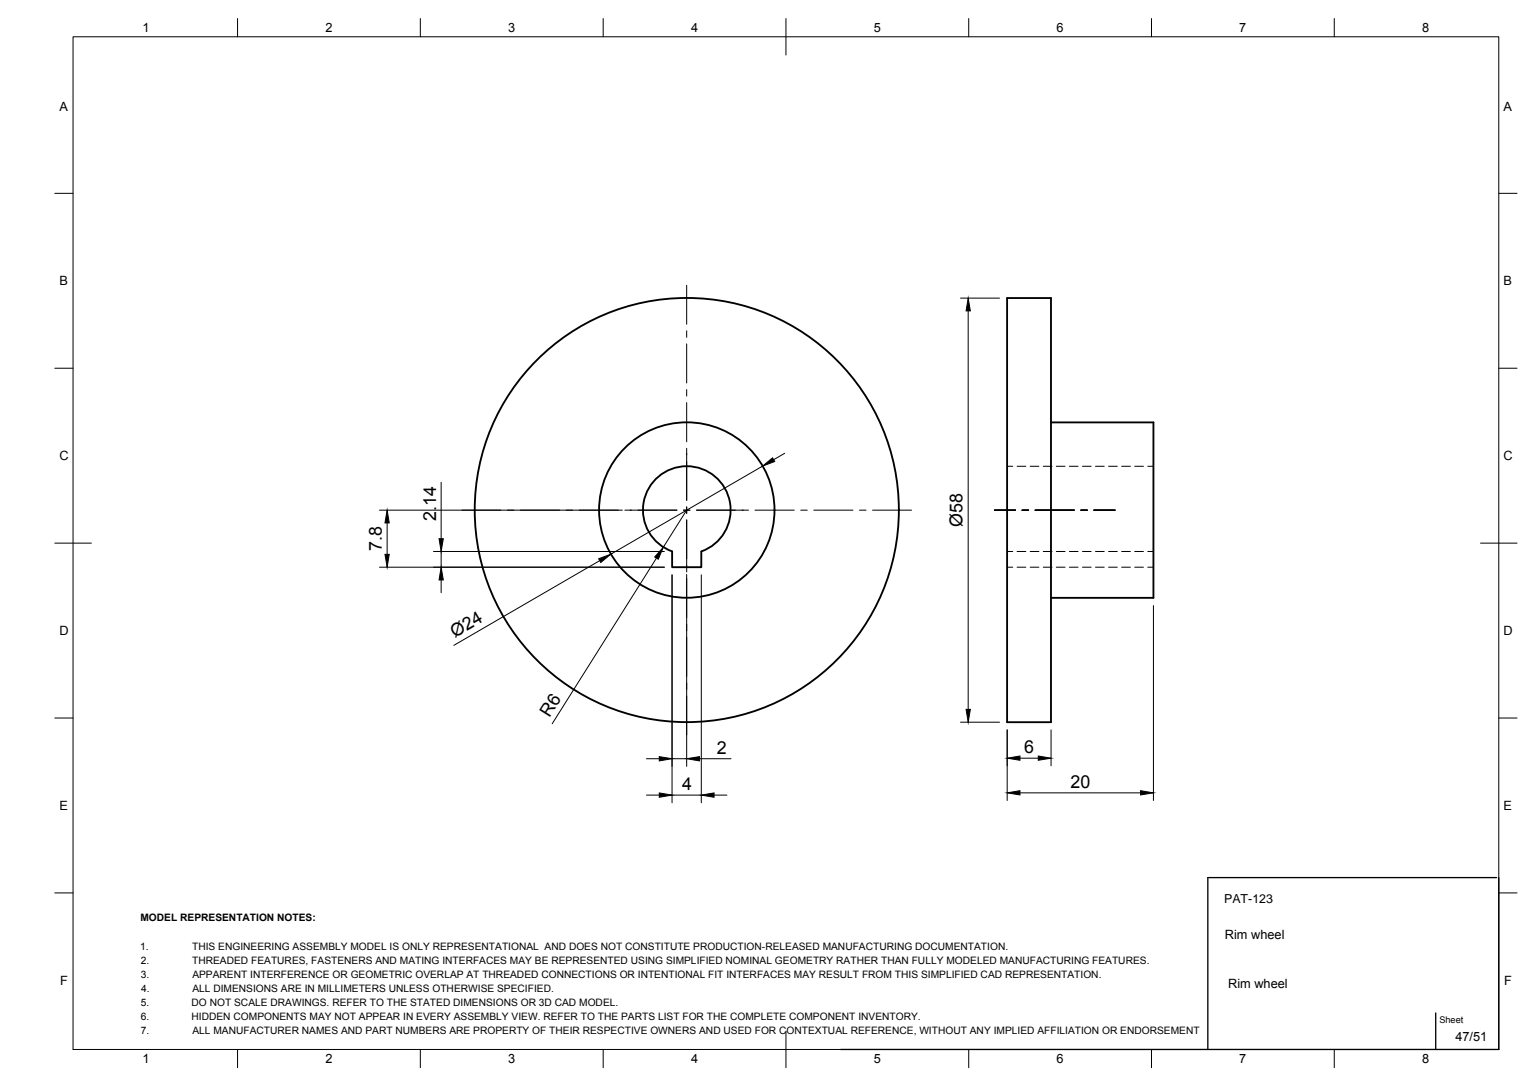
ISO-10303-21;
HEADER;
/* Generated by software containing ST-Developer
 * from STEP Tools, Inc. (www.steptools.com) 
 */

FILE_DESCRIPTION(
/* description */ ('Worm-less right-angle friction wheel drive'),
/* implementation_level */ '2;1');

FILE_NAME(
/* name */ 'Rim wheel.step',
/* time_stamp */ '2026-10-28T03:22:36-07:00',
/* author */ (''),
/* organization */ (''),
/* preprocessor_version */ 'ST-DEVELOPER v20.2',
/* originating_system */ 'Autodesk Translation Framework v15.17.0.0',
/* authorisation */ '');

FILE_SCHEMA (('AUTOMOTIVE_DESIGN { 1 0 10303 214 3 1 1 }'));
ENDSEC;

DATA;
#10=MECHANICAL_DESIGN_GEOMETRIC_PRESENTATION_REPRESENTATION('',(#658),#17046);
#557=SHAPE_REPRESENTATION_RELATIONSHIP('SRR','None',#17303,#604);
#604=ADVANCED_BREP_SHAPE_REPRESENTATION('',(#708),#17039);
#658=STYLED_ITEM('',(#17584),#708);
#708=MANIFOLD_SOLID_BREP('Body1',#8217);
#940=FACE_BOUND('',#2317,.T.);
#941=FACE_BOUND('',#2320,.T.);
#942=FACE_BOUND('',#2324,.T.);
#1171=PLANE('',#9665);
#1172=PLANE('',#9666);
#1173=PLANE('',#9667);
#1174=PLANE('',#9668);
#1175=PLANE('',#9673);
#1176=PLANE('',#9679);
#1622=FACE_OUTER_BOUND('',#2313,.T.);
#1623=FACE_OUTER_BOUND('',#2314,.T.);
#1624=FACE_OUTER_BOUND('',#2315,.T.);
#1625=FACE_OUTER_BOUND('',#2316,.T.);
#1626=FACE_OUTER_BOUND('',#2318,.T.);
#1627=FACE_OUTER_BOUND('',#2319,.T.);
#1628=FACE_OUTER_BOUND('',#2321,.T.);
#1629=FACE_OUTER_BOUND('',#2322,.T.);
#1630=FACE_OUTER_BOUND('',#2323,.T.);
#2313=EDGE_LOOP('',(#7296,#7297,#7298,#7299));
#2314=EDGE_LOOP('',(#7300,#7301,#7302,#7303));
#2315=EDGE_LOOP('',(#7304,#7305,#7306,#7307));
#2316=EDGE_LOOP('',(#7308));
#2317=EDGE_LOOP('',(#7309,#7310,#7311,#7312));
#2318=EDGE_LOOP('',(#7313,#7314,#7315,#7316));
#2319=EDGE_LOOP('',(#7317));
#2320=EDGE_LOOP('',(#7318));
#2321=EDGE_LOOP('',(#7319,#7320,#7321,#7322));
#2322=EDGE_LOOP('',(#7323,#7324,#7325,#7326));
#2323=EDGE_LOOP('',(#7327));
#2324=EDGE_LOOP('',(#7328,#7329,#7330,#7331));
#2843=LINE('',#16561,#3383);
#2844=LINE('',#16563,#3384);
#2845=LINE('',#16565,#3385);
#2846=LINE('',#16566,#3386);
#2847=LINE('',#16569,#3387);
#2848=LINE('',#16571,#3388);
#2849=LINE('',#16572,#3389);
#2850=LINE('',#16575,#3390);
#2851=LINE('',#16577,#3391);
#2852=LINE('',#16578,#3392);
#2853=LINE('',#16592,#3393);
#2854=LINE('',#16595,#3394);
#3383=VECTOR('',#12087,1.);
#3384=VECTOR('',#12088,1.);
#3385=VECTOR('',#12089,1.);
#3386=VECTOR('',#12090,1.);
#3387=VECTOR('',#12093,1.);
#3388=VECTOR('',#12094,1.);
#3389=VECTOR('',#12095,1.);
#3390=VECTOR('',#12098,1.);
#3391=VECTOR('',#12099,1.);
#3392=VECTOR('',#12100,1.);
#3393=VECTOR('',#12119,2.9);
#3394=VECTOR('',#12124,1.2);
#3840=CIRCLE('',#9669,1.2);
#3841=CIRCLE('',#9670,0.6);
#3842=CIRCLE('',#9672,0.6);
#3843=CIRCLE('',#9674,2.9);
#3844=CIRCLE('',#9675,1.2);
#3845=CIRCLE('',#9677,2.9);
#4459=VERTEX_POINT('',#16559);
#4460=VERTEX_POINT('',#16560);
#4461=VERTEX_POINT('',#16562);
#4462=VERTEX_POINT('',#16564);
#4463=VERTEX_POINT('',#16568);
#4464=VERTEX_POINT('',#16570);
#4465=VERTEX_POINT('',#16574);
#4466=VERTEX_POINT('',#16576);
#4467=VERTEX_POINT('',#16580);
#4468=VERTEX_POINT('',#16586);
#4469=VERTEX_POINT('',#16588);
#4470=VERTEX_POINT('',#16591);
#5417=EDGE_CURVE('',#4459,#4460,#2843,.T.);
#5418=EDGE_CURVE('',#4459,#4461,#2844,.T.);
#5419=EDGE_CURVE('',#4462,#4461,#2845,.T.);
#5420=EDGE_CURVE('',#4460,#4462,#2846,.T.);
#5421=EDGE_CURVE('',#4463,#4459,#2847,.T.);
#5422=EDGE_CURVE('',#4463,#4464,#2848,.T.);
#5423=EDGE_CURVE('',#4461,#4464,#2849,.T.);
#5424=EDGE_CURVE('',#4465,#4463,#2850,.T.);
#5425=EDGE_CURVE('',#4466,#4465,#2851,.T.);
#5426=EDGE_CURVE('',#4464,#4466,#2852,.T.);
#5427=EDGE_CURVE('',#4467,#4467,#3840,.T.);
#5428=EDGE_CURVE('',#4466,#4462,#3841,.T.);
#5429=EDGE_CURVE('',#4465,#4460,#3842,.T.);
#5430=EDGE_CURVE('',#4468,#4468,#3843,.T.);
#5431=EDGE_CURVE('',#4469,#4469,#3844,.T.);
#5432=EDGE_CURVE('',#4468,#4470,#2853,.T.);
#5433=EDGE_CURVE('',#4470,#4470,#3845,.T.);
#5434=EDGE_CURVE('',#4467,#4469,#2854,.T.);
#7296=ORIENTED_EDGE('',*,*,#5417,.F.);
#7297=ORIENTED_EDGE('',*,*,#5418,.T.);
#7298=ORIENTED_EDGE('',*,*,#5419,.F.);
#7299=ORIENTED_EDGE('',*,*,#5420,.F.);
#7300=ORIENTED_EDGE('',*,*,#5421,.F.);
#7301=ORIENTED_EDGE('',*,*,#5422,.T.);
#7302=ORIENTED_EDGE('',*,*,#5423,.F.);
#7303=ORIENTED_EDGE('',*,*,#5418,.F.);
#7304=ORIENTED_EDGE('',*,*,#5424,.F.);
#7305=ORIENTED_EDGE('',*,*,#5425,.F.);
#7306=ORIENTED_EDGE('',*,*,#5426,.F.);
#7307=ORIENTED_EDGE('',*,*,#5422,.F.);
#7308=ORIENTED_EDGE('',*,*,#5427,.T.);
#7309=ORIENTED_EDGE('',*,*,#5419,.T.);
#7310=ORIENTED_EDGE('',*,*,#5423,.T.);
#7311=ORIENTED_EDGE('',*,*,#5426,.T.);
#7312=ORIENTED_EDGE('',*,*,#5428,.T.);
#7313=ORIENTED_EDGE('',*,*,#5420,.T.);
#7314=ORIENTED_EDGE('',*,*,#5428,.F.);
#7315=ORIENTED_EDGE('',*,*,#5425,.T.);
#7316=ORIENTED_EDGE('',*,*,#5429,.T.);
#7317=ORIENTED_EDGE('',*,*,#5430,.T.);
#7318=ORIENTED_EDGE('',*,*,#5431,.F.);
#7319=ORIENTED_EDGE('',*,*,#5430,.F.);
#7320=ORIENTED_EDGE('',*,*,#5432,.T.);
#7321=ORIENTED_EDGE('',*,*,#5433,.T.);
#7322=ORIENTED_EDGE('',*,*,#5432,.F.);
#7323=ORIENTED_EDGE('',*,*,#5427,.F.);
#7324=ORIENTED_EDGE('',*,*,#5434,.T.);
#7325=ORIENTED_EDGE('',*,*,#5431,.T.);
#7326=ORIENTED_EDGE('',*,*,#5434,.F.);
#7327=ORIENTED_EDGE('',*,*,#5433,.F.);
#7328=ORIENTED_EDGE('',*,*,#5417,.T.);
#7329=ORIENTED_EDGE('',*,*,#5429,.F.);
#7330=ORIENTED_EDGE('',*,*,#5424,.T.);
#7331=ORIENTED_EDGE('',*,*,#5421,.T.);
#7686=CYLINDRICAL_SURFACE('',#9671,0.6);
#7687=CYLINDRICAL_SURFACE('',#9676,2.9);
#7688=CYLINDRICAL_SURFACE('',#9678,1.2);
#8114=ADVANCED_FACE('',(#1622),#1171,.F.);
#8115=ADVANCED_FACE('',(#1623),#1172,.F.);
#8116=ADVANCED_FACE('',(#1624),#1173,.F.);
#8117=ADVANCED_FACE('',(#1625,#940),#1174,.T.);
#8118=ADVANCED_FACE('',(#1626),#7686,.F.);
#8119=ADVANCED_FACE('',(#1627,#941),#1175,.T.);
#8120=ADVANCED_FACE('',(#1628),#7687,.T.);
#8121=ADVANCED_FACE('',(#1629),#7688,.T.);
#8122=ADVANCED_FACE('',(#1630,#942),#1176,.F.);
#8217=CLOSED_SHELL('',(#8114,#8115,#8116,#8117,#8118,#8119,#8120,#8121,
#8122));
#9664=AXIS2_PLACEMENT_3D('',#16557,#12083,#12084);
#9665=AXIS2_PLACEMENT_3D('',#16558,#12085,#12086);
#9666=AXIS2_PLACEMENT_3D('',#16567,#12091,#12092);
#9667=AXIS2_PLACEMENT_3D('',#16573,#12096,#12097);
#9668=AXIS2_PLACEMENT_3D('',#16579,#12101,#12102);
#9669=AXIS2_PLACEMENT_3D('',#16581,#12103,#12104);
#9670=AXIS2_PLACEMENT_3D('',#16582,#12105,#12106);
#9671=AXIS2_PLACEMENT_3D('',#16583,#12107,#12108);
#9672=AXIS2_PLACEMENT_3D('',#16584,#12109,#12110);
#9673=AXIS2_PLACEMENT_3D('',#16585,#12111,#12112);
#9674=AXIS2_PLACEMENT_3D('',#16587,#12113,#12114);
#9675=AXIS2_PLACEMENT_3D('',#16589,#12115,#12116);
#9676=AXIS2_PLACEMENT_3D('',#16590,#12117,#12118);
#9677=AXIS2_PLACEMENT_3D('',#16593,#12120,#12121);
#9678=AXIS2_PLACEMENT_3D('',#16594,#12122,#12123);
#9679=AXIS2_PLACEMENT_3D('',#16596,#12125,#12126);
#12083=DIRECTION('axis',(0.,0.,1.));
#12084=DIRECTION('refdir',(1.,0.,0.));
#12085=DIRECTION('center_axis',(0.,1.,0.));
#12086=DIRECTION('ref_axis',(0.,0.,1.));
#12087=DIRECTION('',(0.,0.,1.));
#12088=DIRECTION('',(1.,0.,0.));
#12089=DIRECTION('',(0.,0.,-1.));
#12090=DIRECTION('',(1.,0.,0.));
#12091=DIRECTION('center_axis',(0.,0.,-1.));
#12092=DIRECTION('ref_axis',(0.,1.,0.));
#12093=DIRECTION('',(0.,1.,0.));
#12094=DIRECTION('',(1.,0.,0.));
#12095=DIRECTION('',(0.,-1.,0.));
#12096=DIRECTION('center_axis',(0.,-1.,0.));
#12097=DIRECTION('ref_axis',(0.,0.,-1.));
#12098=DIRECTION('',(0.,0.,-1.));
#12099=DIRECTION('',(-1.,0.,0.));
#12100=DIRECTION('',(0.,0.,1.));
#12101=DIRECTION('center_axis',(1.,0.,0.));
#12102=DIRECTION('ref_axis',(0.,0.,-1.));
#12103=DIRECTION('center_axis',(1.,0.,0.));
#12104=DIRECTION('ref_axis',(0.,0.,-1.));
#12105=DIRECTION('center_axis',(-1.,0.,0.));
#12106=DIRECTION('ref_axis',(0.,0.,-1.));
#12107=DIRECTION('center_axis',(1.,0.,0.));
#12108=DIRECTION('ref_axis',(0.,1.22464679914735E-16,1.));
#12109=DIRECTION('center_axis',(-1.,0.,0.));
#12110=DIRECTION('ref_axis',(0.,0.,-1.));
#12111=DIRECTION('center_axis',(1.,0.,0.));
#12112=DIRECTION('ref_axis',(0.,0.,-1.));
#12113=DIRECTION('center_axis',(1.,0.,0.));
#12114=DIRECTION('ref_axis',(0.,0.,-1.));
#12115=DIRECTION('center_axis',(1.,0.,0.));
#12116=DIRECTION('ref_axis',(0.,0.,-1.));
#12117=DIRECTION('center_axis',(1.,0.,0.));
#12118=DIRECTION('ref_axis',(0.,0.,-1.));
#12119=DIRECTION('',(-1.,0.,0.));
#12120=DIRECTION('center_axis',(1.,0.,0.));
#12121=DIRECTION('ref_axis',(0.,0.,-1.));
#12122=DIRECTION('center_axis',(1.,0.,0.));
#12123=DIRECTION('ref_axis',(0.,0.,-1.));
#12124=DIRECTION('',(-1.,0.,0.));
#12125=DIRECTION('center_axis',(1.,0.,0.));
#12126=DIRECTION('ref_axis',(0.,0.,-1.));
#16557=CARTESIAN_POINT('',(0.,0.,0.));
#16558=CARTESIAN_POINT('Origin',(1.1,3.2,6.22));
#16559=CARTESIAN_POINT('',(1.2,3.2,6.22));
#16560=CARTESIAN_POINT('',(1.2,3.2,6.43431457505076));
#16561=CARTESIAN_POINT('',(1.2,3.2,6.61));
#16562=CARTESIAN_POINT('',(3.2,3.2,6.22));
#16563=CARTESIAN_POINT('',(1.1,3.2,6.22));
#16564=CARTESIAN_POINT('',(3.2,3.2,6.43431457505076));
#16565=CARTESIAN_POINT('',(3.2,3.2,6.61));
#16566=CARTESIAN_POINT('',(1.2,3.2,6.43431457505076));
#16567=CARTESIAN_POINT('Origin',(1.1,2.8,6.22));
#16568=CARTESIAN_POINT('',(1.2,2.8,6.22));
#16569=CARTESIAN_POINT('',(1.2,2.9,6.22));
#16570=CARTESIAN_POINT('',(3.2,2.8,6.22));
#16571=CARTESIAN_POINT('',(1.1,2.8,6.22));
#16572=CARTESIAN_POINT('',(3.2,2.9,6.22));
#16573=CARTESIAN_POINT('Origin',(1.1,2.8,7.));
#16574=CARTESIAN_POINT('',(1.2,2.8,6.43431457505076));
#16575=CARTESIAN_POINT('',(1.2,2.8,7.));
#16576=CARTESIAN_POINT('',(3.2,2.8,6.43431457505076));
#16577=CARTESIAN_POINT('',(1.2,2.8,6.43431457505076));
#16578=CARTESIAN_POINT('',(3.2,2.8,7.));
#16579=CARTESIAN_POINT('Origin',(3.2,3.,7.));
#16580=CARTESIAN_POINT('',(3.2,3.,8.2));
#16581=CARTESIAN_POINT('Origin',(3.2,3.,7.));
#16582=CARTESIAN_POINT('Origin',(3.2,3.,7.));
#16583=CARTESIAN_POINT('Origin',(1.2,3.,7.));
#16584=CARTESIAN_POINT('Origin',(1.2,3.,7.));
#16585=CARTESIAN_POINT('Origin',(1.8,3.,7.));
#16586=CARTESIAN_POINT('',(1.8,3.,9.9));
#16587=CARTESIAN_POINT('Origin',(1.8,3.,7.));
#16588=CARTESIAN_POINT('',(1.8,3.,8.2));
#16589=CARTESIAN_POINT('Origin',(1.8,3.,7.));
#16590=CARTESIAN_POINT('Origin',(1.2,3.,7.));
#16591=CARTESIAN_POINT('',(1.2,3.,9.9));
#16592=CARTESIAN_POINT('',(1.2,3.,9.9));
#16593=CARTESIAN_POINT('Origin',(1.2,3.,7.));
#16594=CARTESIAN_POINT('Origin',(1.2,3.,7.));
#16595=CARTESIAN_POINT('',(1.2,3.,8.2));
#16596=CARTESIAN_POINT('Origin',(1.2,3.,7.));
#16986=UNCERTAINTY_MEASURE_WITH_UNIT(LENGTH_MEASURE(0.001),#17047,
'DISTANCE_ACCURACY_VALUE',
'Maximum model space distance between geometric entities at asserted c
onnectivities');
#16993=UNCERTAINTY_MEASURE_WITH_UNIT(LENGTH_MEASURE(0.001),#17047,
'DISTANCE_ACCURACY_VALUE',
'Maximum model space distance between geometric entities at asserted c
onnectivities');
#17039=(
GEOMETRIC_REPRESENTATION_CONTEXT(3)
GLOBAL_UNCERTAINTY_ASSIGNED_CONTEXT((#16986))
GLOBAL_UNIT_ASSIGNED_CONTEXT((#17047,#17049,#17050))
REPRESENTATION_CONTEXT('','3D')
);
#17046=(
GEOMETRIC_REPRESENTATION_CONTEXT(3)
GLOBAL_UNCERTAINTY_ASSIGNED_CONTEXT((#16993))
GLOBAL_UNIT_ASSIGNED_CONTEXT((#17047,#17049,#17050))
REPRESENTATION_CONTEXT('','3D')
);
#17047=(
LENGTH_UNIT()
NAMED_UNIT(*)
SI_UNIT(.CENTI.,.METRE.)
);
#17049=(
NAMED_UNIT(*)
PLANE_ANGLE_UNIT()
SI_UNIT($,.RADIAN.)
);
#17050=(
NAMED_UNIT(*)
SI_UNIT($,.STERADIAN.)
SOLID_ANGLE_UNIT()
);
#17096=SHAPE_DEFINITION_REPRESENTATION(#17230,#17303);
#17230=PRODUCT_DEFINITION_SHAPE('',$,#17356);
#17303=SHAPE_REPRESENTATION('',(#9664),#17039);
#17310=PRODUCT_DEFINITION_CONTEXT('part definition',#17468,'design');
#17356=PRODUCT_DEFINITION('Rim wheel','Rim wheel',#17408,#17310);
#17408=PRODUCT_DEFINITION_FORMATION('',$,#17515);
#17468=APPLICATION_CONTEXT(
'Core Data for Automotive Mechanical Design Process');
#17469=PRODUCT_CONTEXT('part definition',#17468,'mechanical');
#17515=PRODUCT('Rim wheel','Rim wheel','Rim wheel',(#17469));
#17578=COLOUR_RGB('Sky Blue',0.24,0.69,0.87);
#17579=FILL_AREA_STYLE_COLOUR('',#17578);
#17580=FILL_AREA_STYLE('',(#17579));
#17581=SURFACE_STYLE_FILL_AREA(#17580);
#17582=SURFACE_SIDE_STYLE('',(#17581));
#17583=SURFACE_STYLE_USAGE(.BOTH.,#17582);
#17584=PRESENTATION_STYLE_ASSIGNMENT((#17583));
ENDSEC;
END-ISO-10303-21;
